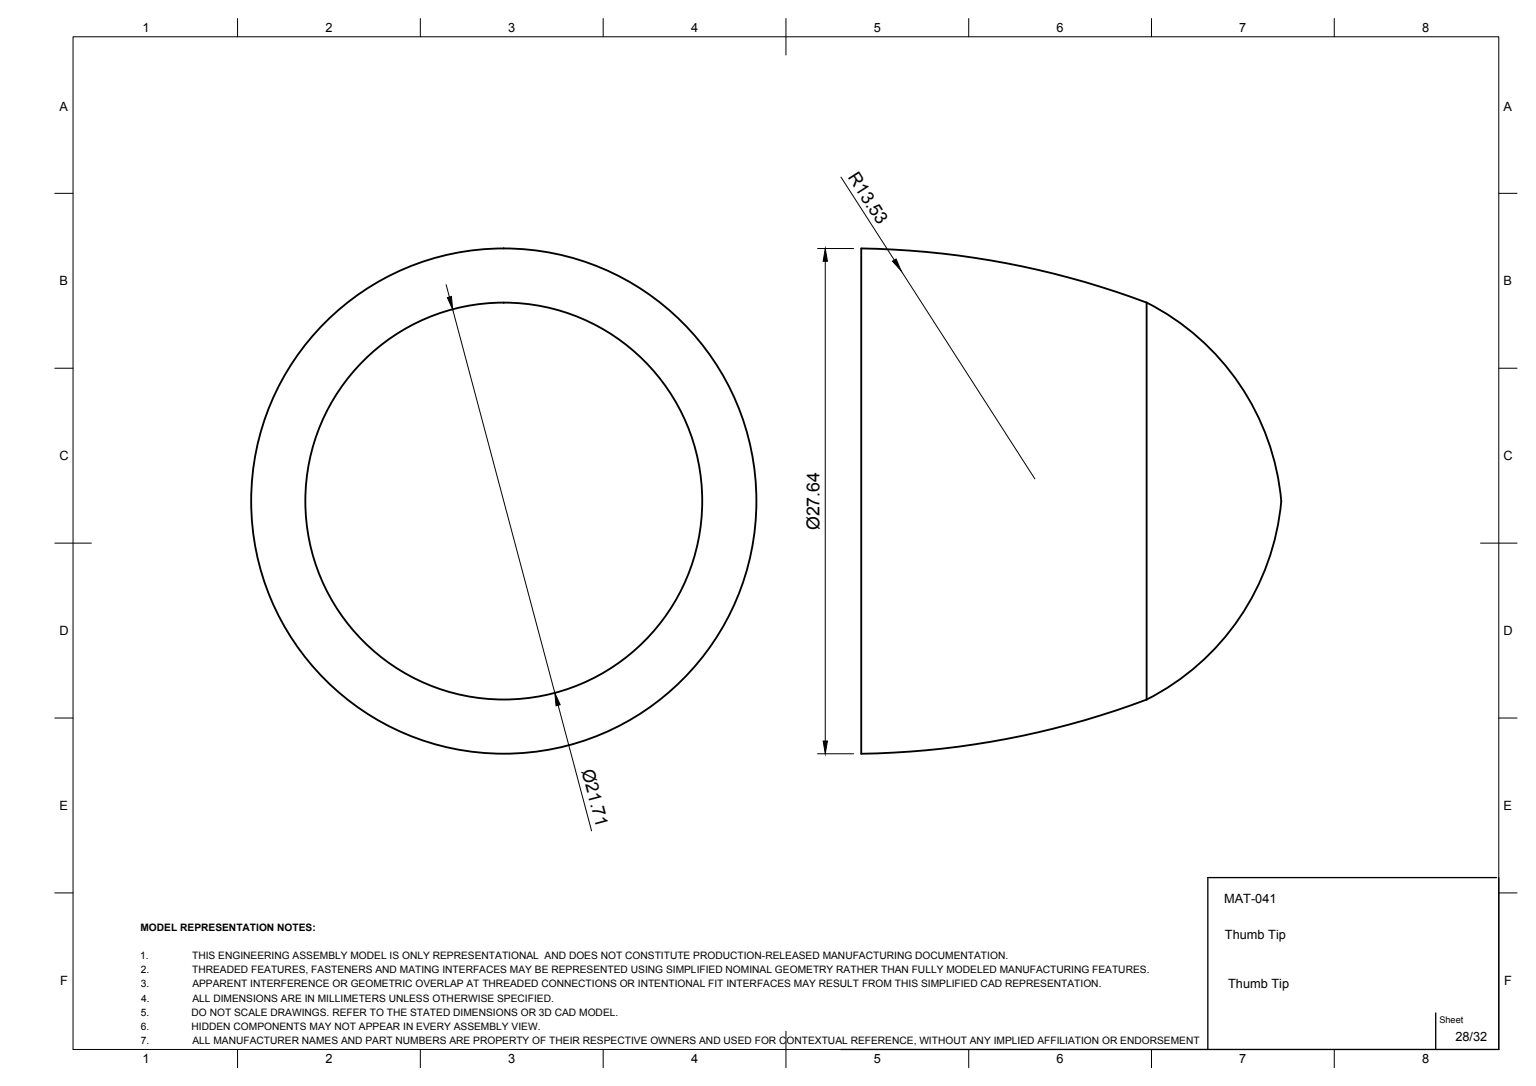
ISO-10303-21;
HEADER;
/* Generated by software containing ST-Developer
 * from STEP Tools, Inc. (www.steptools.com) 
 */

FILE_DESCRIPTION(
/* description */ ('STEP AP214'),
/* implementation_level */ '2;1');

FILE_NAME(
/* name */ 'Thumb Tip.step',
/* time_stamp */ '2026-11-14T21:57:47-08:00',
/* author */ (''),
/* organization */ (''),
/* preprocessor_version */ 'ST-DEVELOPER v20.2',
/* originating_system */ 'Autodesk Translation Framework v15.17.0.0',
/* authorisation */ '');

FILE_SCHEMA (('AUTOMOTIVE_DESIGN { 1 0 10303 214 3 1 1 }'));
ENDSEC;

DATA;
#10=MECHANICAL_DESIGN_GEOMETRIC_PRESENTATION_REPRESENTATION('',(#263),#13199);
#19=(
BOUNDED_SURFACE()
B_SPLINE_SURFACE(2,2,((#12988,#12989,#12990,#12991,#12992,#12993,#12994,
#12995,#12996),(#12997,#12998,#12999,#13000,#13001,#13002,#13003,#13004,
#13005),(#13006,#13007,#13008,#13009,#13010,#13011,#13012,#13013,#13014)),
 .UNSPECIFIED.,.F.,.T.,.F.)
B_SPLINE_SURFACE_WITH_KNOTS((3,3),(3,2,2,2,3),(-1.48074001480244,-0.468405301545521),
(-3.14159265358979,-1.5707963267949,0.,1.5707963267949,3.14159265358979),
 .UNSPECIFIED.)
GEOMETRIC_REPRESENTATION_ITEM()
RATIONAL_B_SPLINE_SURFACE(((1.,0.707106781186548,1.,0.707106781186548,1.,
0.707106781186548,1.,0.707106781186548,1.),(0.874609102422644,0.618442027210531,
0.874609102422644,0.618442027210531,0.874609102422644,0.618442027210531,
0.874609102422644,0.618442027210531,0.874609102422644),(1.,0.707106781186548,
1.,0.707106781186548,1.,0.707106781186548,1.,0.707106781186548,1.)))
REPRESENTATION_ITEM('')
SURFACE()
);
#20=(
BOUNDED_SURFACE()
B_SPLINE_SURFACE(2,2,((#13019,#13020,#13021,#13022,#13023,#13024,#13025,
#13026,#13027),(#13028,#13029,#13030,#13031,#13032,#13033,#13034,#13035,
#13036),(#13037,#13038,#13039,#13040,#13041,#13042,#13043,#13044,#13045)),
 .UNSPECIFIED.,.F.,.T.,.F.)
B_SPLINE_SURFACE_WITH_KNOTS((3,3),(3,2,2,2,3),(-0.359971068140638,-0.0153537783592699),
(-3.14159265358979,-1.5707963267949,0.,1.5707963267949,3.14159265358979),
 .UNSPECIFIED.)
GEOMETRIC_REPRESENTATION_ITEM()
RATIONAL_B_SPLINE_SURFACE(((1.,0.707106781186548,1.,0.707106781186548,1.,
0.707106781186548,1.,0.707106781186548,1.),(0.985191558786762,0.696635631985865,
0.985191558786762,0.696635631985865,0.985191558786762,0.696635631985865,
0.985191558786762,0.696635631985865,0.985191558786762),(1.,0.707106781186548,
1.,0.707106781186548,1.,0.707106781186548,1.,0.707106781186548,1.)))
REPRESENTATION_ITEM('')
SURFACE()
);
#227=SHAPE_REPRESENTATION_RELATIONSHIP('SRR','None',#13299,#245);
#245=ADVANCED_BREP_SHAPE_REPRESENTATION('',(#281),#13195);
#263=STYLED_ITEM('',(#13409),#281);
#281=MANIFOLD_SOLID_BREP('Body1',#6858);
#596=PLANE('',#7781);
#2168=FACE_OUTER_BOUND('',#2651,.T.);
#2169=FACE_OUTER_BOUND('',#2652,.T.);
#2170=FACE_OUTER_BOUND('',#2653,.T.);
#2651=EDGE_LOOP('',(#6356,#6357,#6358));
#2652=EDGE_LOOP('',(#6359,#6360,#6361,#6362));
#2653=EDGE_LOOP('',(#6363));
#2982=CIRCLE('',#7777,10.8559587775082);
#2983=CIRCLE('',#7778,13.5301235990631);
#2984=CIRCLE('',#7779,13.82);
#2985=CIRCLE('',#7780,46.3311569126792);
#3587=VERTEX_POINT('',#13015);
#3588=VERTEX_POINT('',#13017);
#3589=VERTEX_POINT('',#13046);
#4515=EDGE_CURVE('',#3587,#3587,#2982,.T.);
#4516=EDGE_CURVE('',#3587,#3588,#2983,.T.);
#4517=EDGE_CURVE('',#3589,#3589,#2984,.T.);
#4518=EDGE_CURVE('',#3589,#3587,#2985,.T.);
#6356=ORIENTED_EDGE('',*,*,#4515,.F.);
#6357=ORIENTED_EDGE('',*,*,#4516,.T.);
#6358=ORIENTED_EDGE('',*,*,#4516,.F.);
#6359=ORIENTED_EDGE('',*,*,#4517,.F.);
#6360=ORIENTED_EDGE('',*,*,#4518,.T.);
#6361=ORIENTED_EDGE('',*,*,#4515,.T.);
#6362=ORIENTED_EDGE('',*,*,#4518,.F.);
#6363=ORIENTED_EDGE('',*,*,#4517,.T.);
#6820=ADVANCED_FACE('',(#2168),#19,.F.);
#6821=ADVANCED_FACE('',(#2169),#20,.F.);
#6822=ADVANCED_FACE('',(#2170),#596,.T.);
#6858=CLOSED_SHELL('',(#6820,#6821,#6822));
#7776=AXIS2_PLACEMENT_3D('',#12987,#9754,#9755);
#7777=AXIS2_PLACEMENT_3D('',#13016,#9756,#9757);
#7778=AXIS2_PLACEMENT_3D('',#13018,#9758,#9759);
#7779=AXIS2_PLACEMENT_3D('',#13047,#9760,#9761);
#7780=AXIS2_PLACEMENT_3D('',#13048,#9762,#9763);
#7781=AXIS2_PLACEMENT_3D('',#13049,#9764,#9765);
#9754=DIRECTION('axis',(0.,0.,1.));
#9755=DIRECTION('refdir',(1.,0.,0.));
#9756=DIRECTION('center_axis',(0.,-1.,0.));
#9757=DIRECTION('ref_axis',(0.,0.,-1.));
#9758=DIRECTION('center_axis',(-1.,0.,-1.22464679914735E-16));
#9759=DIRECTION('ref_axis',(-1.22464679914735E-16,0.,1.));
#9760=DIRECTION('center_axis',(0.,-1.,0.));
#9761=DIRECTION('ref_axis',(0.,0.,-1.));
#9762=DIRECTION('center_axis',(-1.,0.,-1.22464679914735E-16));
#9763=DIRECTION('ref_axis',(-1.22464679914735E-16,0.,1.));
#9764=DIRECTION('center_axis',(0.,-1.,0.));
#9765=DIRECTION('ref_axis',(0.,0.,-1.));
#12987=CARTESIAN_POINT('',(0.,0.,0.));
#12988=CARTESIAN_POINT('Ctrl Pts',(0.,22.9756202217091,1.38777878078145E-15));
#12989=CARTESIAN_POINT('Ctrl Pts',(-1.38777878078145E-15,22.9756202217091,
1.38777878078145E-15));
#12990=CARTESIAN_POINT('Ctrl Pts',(-1.38777878078145E-15,22.9756202217091,
0.));
#12991=CARTESIAN_POINT('Ctrl Pts',(-1.38777878078145E-15,22.9756202217091,
-1.38777878078145E-15));
#12992=CARTESIAN_POINT('Ctrl Pts',(0.,22.9756202217091,-1.38777878078145E-15));
#12993=CARTESIAN_POINT('Ctrl Pts',(1.38777878078145E-15,22.9756202217091,
-1.38777878078145E-15));
#12994=CARTESIAN_POINT('Ctrl Pts',(1.38777878078145E-15,22.9756202217091,
0.));
#12995=CARTESIAN_POINT('Ctrl Pts',(1.38777878078145E-15,22.9756202217091,
1.38777878078145E-15));
#12996=CARTESIAN_POINT('Ctrl Pts',(0.,22.9756202217091,1.38777878078145E-15));
#12997=CARTESIAN_POINT('Ctrl Pts',(0.,22.3010873717989,7.46986335401695));
#12998=CARTESIAN_POINT('Ctrl Pts',(-7.46986335401695,22.3010873717989,7.46986335401695));
#12999=CARTESIAN_POINT('Ctrl Pts',(-7.46986335401695,22.3010873717989,0.));
#13000=CARTESIAN_POINT('Ctrl Pts',(-7.46986335401695,22.3010873717989,-7.46986335401695));
#13001=CARTESIAN_POINT('Ctrl Pts',(0.,22.3010873717989,-7.46986335401695));
#13002=CARTESIAN_POINT('Ctrl Pts',(7.46986335401695,22.3010873717989,-7.46986335401695));
#13003=CARTESIAN_POINT('Ctrl Pts',(7.46986335401695,22.3010873717989,0.));
#13004=CARTESIAN_POINT('Ctrl Pts',(7.46986335401695,22.3010873717989,7.46986335401695));
#13005=CARTESIAN_POINT('Ctrl Pts',(0.,22.3010873717989,7.46986335401695));
#13006=CARTESIAN_POINT('Ctrl Pts',(0.,15.6086878860909,10.8559587775082));
#13007=CARTESIAN_POINT('Ctrl Pts',(-10.8559587775082,15.6086878860909,10.8559587775082));
#13008=CARTESIAN_POINT('Ctrl Pts',(-10.8559587775082,15.6086878860909,0.));
#13009=CARTESIAN_POINT('Ctrl Pts',(-10.8559587775082,15.6086878860909,-10.8559587775082));
#13010=CARTESIAN_POINT('Ctrl Pts',(0.,15.6086878860909,-10.8559587775082));
#13011=CARTESIAN_POINT('Ctrl Pts',(10.8559587775082,15.6086878860909,-10.8559587775082));
#13012=CARTESIAN_POINT('Ctrl Pts',(10.8559587775082,15.6086878860909,0.));
#13013=CARTESIAN_POINT('Ctrl Pts',(10.8559587775082,15.6086878860909,10.8559587775082));
#13014=CARTESIAN_POINT('Ctrl Pts',(0.,15.6086878860909,10.8559587775082));
#13015=CARTESIAN_POINT('',(1.51096669663837E-15,15.6086878860909,10.8559587775082));
#13016=CARTESIAN_POINT('Origin',(0.,15.6086878860909,0.));
#13017=CARTESIAN_POINT('',(1.30104260698261E-15,22.9756202217091,0.));
#13018=CARTESIAN_POINT('Origin',(1.49018292596266E-16,9.50032514580282,
-1.21682670219706));
#13019=CARTESIAN_POINT('Ctrl Pts',(0.,15.6086878860909,10.8559587775082));
#13020=CARTESIAN_POINT('Ctrl Pts',(-10.8559587775082,15.6086878860909,10.8559587775082));
#13021=CARTESIAN_POINT('Ctrl Pts',(-10.8559587775082,15.6086878860909,0.));
#13022=CARTESIAN_POINT('Ctrl Pts',(-10.8559587775082,15.6086878860909,-10.8559587775082));
#13023=CARTESIAN_POINT('Ctrl Pts',(0.,15.6086878860909,-10.8559587775082));
#13024=CARTESIAN_POINT('Ctrl Pts',(10.8559587775082,15.6086878860909,-10.8559587775082));
#13025=CARTESIAN_POINT('Ctrl Pts',(10.8559587775082,15.6086878860909,0.));
#13026=CARTESIAN_POINT('Ctrl Pts',(10.8559587775082,15.6086878860909,10.8559587775082));
#13027=CARTESIAN_POINT('Ctrl Pts',(0.,15.6086878860909,10.8559587775082));
#13028=CARTESIAN_POINT('Ctrl Pts',(0.,8.06226657049109,13.6962040180237));
#13029=CARTESIAN_POINT('Ctrl Pts',(-13.6962040180237,8.06226657049109,13.6962040180237));
#13030=CARTESIAN_POINT('Ctrl Pts',(-13.6962040180237,8.06226657049109,0.));
#13031=CARTESIAN_POINT('Ctrl Pts',(-13.6962040180237,8.06226657049109,-13.6962040180237));
#13032=CARTESIAN_POINT('Ctrl Pts',(0.,8.06226657049109,-13.6962040180237));
#13033=CARTESIAN_POINT('Ctrl Pts',(13.6962040180237,8.06226657049109,-13.6962040180237));
#13034=CARTESIAN_POINT('Ctrl Pts',(13.6962040180237,8.06226657049109,0.));
#13035=CARTESIAN_POINT('Ctrl Pts',(13.6962040180237,8.06226657049109,13.6962040180237));
#13036=CARTESIAN_POINT('Ctrl Pts',(0.,8.06226657049109,13.6962040180237));
#13037=CARTESIAN_POINT('Ctrl Pts',(0.,0.,13.82));
#13038=CARTESIAN_POINT('Ctrl Pts',(-13.82,0.,13.82));
#13039=CARTESIAN_POINT('Ctrl Pts',(-13.82,0.,0.));
#13040=CARTESIAN_POINT('Ctrl Pts',(-13.82,0.,-13.82));
#13041=CARTESIAN_POINT('Ctrl Pts',(0.,0.,-13.82));
#13042=CARTESIAN_POINT('Ctrl Pts',(13.82,0.,-13.82));
#13043=CARTESIAN_POINT('Ctrl Pts',(13.82,0.,0.));
#13044=CARTESIAN_POINT('Ctrl Pts',(13.82,0.,13.82));
#13045=CARTESIAN_POINT('Ctrl Pts',(0.,0.,13.82));
#13046=CARTESIAN_POINT('',(-1.69246187642164E-15,0.,13.82));
#13047=CARTESIAN_POINT('Origin',(0.,0.,0.));
#13048=CARTESIAN_POINT('Origin',(3.98079965616974E-15,-0.711330365603759,
-32.505696001013));
#13049=CARTESIAN_POINT('Origin',(0.,0.,0.));
#13169=UNCERTAINTY_MEASURE_WITH_UNIT(LENGTH_MEASURE(0.01),#13200,
'DISTANCE_ACCURACY_VALUE',
'Maximum model space distance between geometric entities at asserted c
onnectivities');
#13173=UNCERTAINTY_MEASURE_WITH_UNIT(LENGTH_MEASURE(0.01),#13200,
'DISTANCE_ACCURACY_VALUE',
'Maximum model space distance between geometric entities at asserted c
onnectivities');
#13195=(
GEOMETRIC_REPRESENTATION_CONTEXT(3)
GLOBAL_UNCERTAINTY_ASSIGNED_CONTEXT((#13169))
GLOBAL_UNIT_ASSIGNED_CONTEXT((#13200,#13202,#13203))
REPRESENTATION_CONTEXT('','3D')
);
#13199=(
GEOMETRIC_REPRESENTATION_CONTEXT(3)
GLOBAL_UNCERTAINTY_ASSIGNED_CONTEXT((#13173))
GLOBAL_UNIT_ASSIGNED_CONTEXT((#13200,#13202,#13203))
REPRESENTATION_CONTEXT('','3D')
);
#13200=(
LENGTH_UNIT()
NAMED_UNIT(*)
SI_UNIT(.MILLI.,.METRE.)
);
#13202=(
NAMED_UNIT(*)
PLANE_ANGLE_UNIT()
SI_UNIT($,.RADIAN.)
);
#13203=(
NAMED_UNIT(*)
SI_UNIT($,.STERADIAN.)
SOLID_ANGLE_UNIT()
);
#13225=SHAPE_DEFINITION_REPRESENTATION(#13264,#13299);
#13264=PRODUCT_DEFINITION_SHAPE('',$,#13325);
#13299=SHAPE_REPRESENTATION('',(#7776),#13195);
#13303=PRODUCT_DEFINITION_CONTEXT('part definition',#13380,'design');
#13325=PRODUCT_DEFINITION('Thumb Tip','Thumb Tip',#13350,#13303);
#13350=PRODUCT_DEFINITION_FORMATION('',$,#13403);
#13380=APPLICATION_CONTEXT(
'Core Data for Automotive Mechanical Design Process');
#13381=PRODUCT_CONTEXT('part definition',#13380,'mechanical');
#13403=PRODUCT('Thumb Tip','Thumb Tip',$,(#13381));
#13409=PRESENTATION_STYLE_ASSIGNMENT((#13414));
#13414=SURFACE_STYLE_USAGE(.BOTH.,#13419);
#13419=SURFACE_SIDE_STYLE('',(#13424));
#13424=SURFACE_STYLE_FILL_AREA(#13429);
#13429=FILL_AREA_STYLE('Opaque(61,176,222)',(#13434));
#13434=FILL_AREA_STYLE_COLOUR('Opaque(61,176,222)',#13439);
#13439=COLOUR_RGB('Opaque(61,176,222)',0.23921568627451,0.690196078431373,
0.870588235294118);
ENDSEC;
END-ISO-10303-21;
